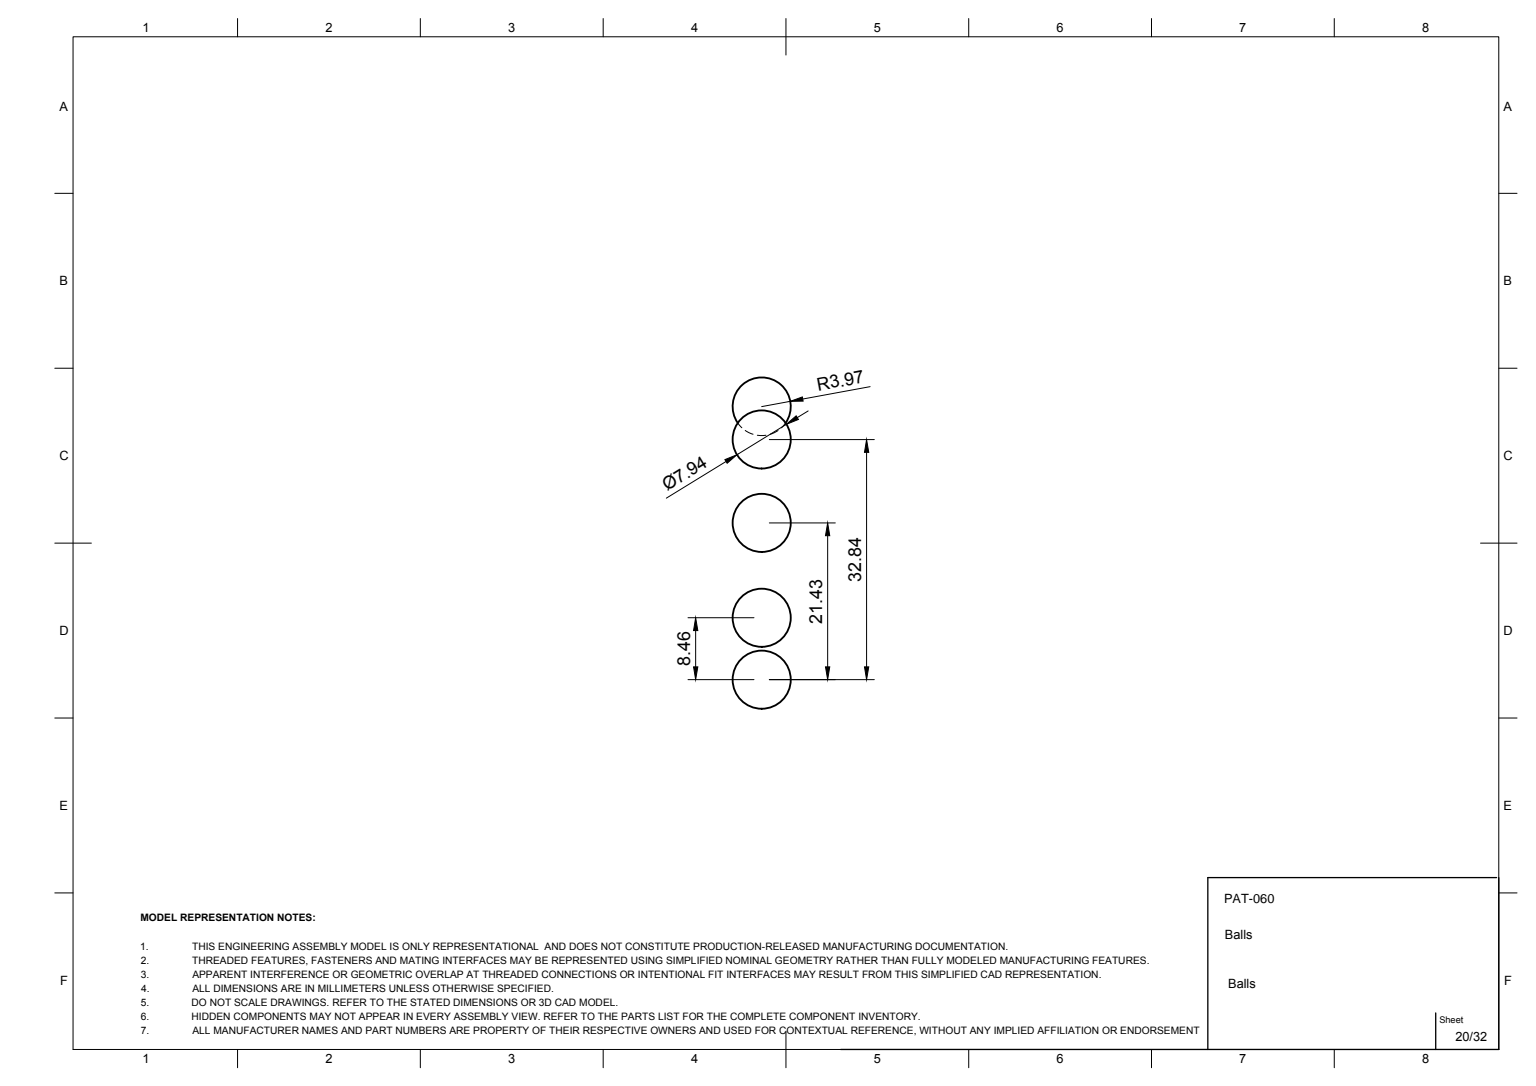
ISO-10303-21;
HEADER;
/* Generated by software containing ST-Developer
 * from STEP Tools, Inc. (www.steptools.com) 
 */

FILE_DESCRIPTION(
/* description */ ('Indexing fixture plate with plunger'),
/* implementation_level */ '2;1');

FILE_NAME(
/* name */ 'Balls.step',
/* time_stamp */ '2026-10-28T03:23:41-07:00',
/* author */ (''),
/* organization */ (''),
/* preprocessor_version */ 'ST-DEVELOPER v20.2',
/* originating_system */ 'Autodesk Translation Framework v15.17.0.0',
/* authorisation */ '');

FILE_SCHEMA (('AUTOMOTIVE_DESIGN { 1 0 10303 214 3 1 1 }'));
ENDSEC;

DATA;
#10=MECHANICAL_DESIGN_GEOMETRIC_PRESENTATION_REPRESENTATION('',(#332,#333,#334,#335,#336,#337,#338,#339,#340),#10020);
#195=SPHERICAL_SURFACE('',#5126,0.3969);
#196=SPHERICAL_SURFACE('',#5128,0.3969);
#197=SPHERICAL_SURFACE('',#5130,0.3969);
#198=SPHERICAL_SURFACE('',#5132,0.3969);
#199=SPHERICAL_SURFACE('',#5134,0.3969);
#200=SPHERICAL_SURFACE('',#5136,0.3969);
#201=SPHERICAL_SURFACE('',#5138,0.3969);
#202=SPHERICAL_SURFACE('',#5140,0.3969);
#203=SPHERICAL_SURFACE('',#5142,0.3969);
#278=SHAPE_REPRESENTATION_RELATIONSHIP('SRR','None',#10153,#305);
#305=ADVANCED_BREP_SHAPE_REPRESENTATION('',(#367,#368,#369,#370,#371,#372,
#373,#374,#375),#10006);
#332=STYLED_ITEM('',(#10368),#367);
#333=STYLED_ITEM('',(#10368),#368);
#334=STYLED_ITEM('',(#10368),#369);
#335=STYLED_ITEM('',(#10368),#370);
#336=STYLED_ITEM('',(#10368),#371);
#337=STYLED_ITEM('',(#10368),#372);
#338=STYLED_ITEM('',(#10368),#373);
#339=STYLED_ITEM('',(#10368),#374);
#340=STYLED_ITEM('',(#10368),#375);
#367=MANIFOLD_SOLID_BREP('Body1',#4587);
#368=MANIFOLD_SOLID_BREP('Body2',#4588);
#369=MANIFOLD_SOLID_BREP('Body3',#4589);
#370=MANIFOLD_SOLID_BREP('Body4',#4590);
#371=MANIFOLD_SOLID_BREP('Body5',#4591);
#372=MANIFOLD_SOLID_BREP('Body6',#4592);
#373=MANIFOLD_SOLID_BREP('Body7',#4593);
#374=MANIFOLD_SOLID_BREP('Body8',#4594);
#375=MANIFOLD_SOLID_BREP('Body9',#4595);
#772=FACE_OUTER_BOUND('',#1106,.T.);
#773=FACE_OUTER_BOUND('',#1107,.T.);
#774=FACE_OUTER_BOUND('',#1108,.T.);
#775=FACE_OUTER_BOUND('',#1109,.T.);
#776=FACE_OUTER_BOUND('',#1110,.T.);
#777=FACE_OUTER_BOUND('',#1111,.T.);
#778=FACE_OUTER_BOUND('',#1112,.T.);
#779=FACE_OUTER_BOUND('',#1113,.T.);
#780=FACE_OUTER_BOUND('',#1114,.T.);
#1106=EDGE_LOOP('',(#3435,#3436));
#1107=EDGE_LOOP('',(#3437,#3438));
#1108=EDGE_LOOP('',(#3439,#3440));
#1109=EDGE_LOOP('',(#3441,#3442));
#1110=EDGE_LOOP('',(#3443,#3444));
#1111=EDGE_LOOP('',(#3445,#3446));
#1112=EDGE_LOOP('',(#3447,#3448));
#1113=EDGE_LOOP('',(#3449,#3450));
#1114=EDGE_LOOP('',(#3451,#3452));
#1931=CIRCLE('',#5127,0.3969);
#1932=CIRCLE('',#5129,0.3969);
#1933=CIRCLE('',#5131,0.3969);
#1934=CIRCLE('',#5133,0.3969);
#1935=CIRCLE('',#5135,0.3969);
#1936=CIRCLE('',#5137,0.3969);
#1937=CIRCLE('',#5139,0.3969);
#1938=CIRCLE('',#5141,0.3969);
#1939=CIRCLE('',#5143,0.3969);
#2257=VERTEX_POINT('',#8670);
#2258=VERTEX_POINT('',#8671);
#2259=VERTEX_POINT('',#8674);
#2260=VERTEX_POINT('',#8675);
#2261=VERTEX_POINT('',#8678);
#2262=VERTEX_POINT('',#8679);
#2263=VERTEX_POINT('',#8682);
#2264=VERTEX_POINT('',#8683);
#2265=VERTEX_POINT('',#8686);
#2266=VERTEX_POINT('',#8687);
#2267=VERTEX_POINT('',#8690);
#2268=VERTEX_POINT('',#8691);
#2269=VERTEX_POINT('',#8694);
#2270=VERTEX_POINT('',#8695);
#2271=VERTEX_POINT('',#8698);
#2272=VERTEX_POINT('',#8699);
#2273=VERTEX_POINT('',#8702);
#2274=VERTEX_POINT('',#8703);
#2697=EDGE_CURVE('',#2257,#2258,#1931,.T.);
#2698=EDGE_CURVE('',#2259,#2260,#1932,.T.);
#2699=EDGE_CURVE('',#2261,#2262,#1933,.T.);
#2700=EDGE_CURVE('',#2263,#2264,#1934,.T.);
#2701=EDGE_CURVE('',#2265,#2266,#1935,.T.);
#2702=EDGE_CURVE('',#2267,#2268,#1936,.T.);
#2703=EDGE_CURVE('',#2269,#2270,#1937,.T.);
#2704=EDGE_CURVE('',#2271,#2272,#1938,.T.);
#2705=EDGE_CURVE('',#2273,#2274,#1939,.T.);
#3435=ORIENTED_EDGE('',*,*,#2697,.T.);
#3436=ORIENTED_EDGE('',*,*,#2697,.F.);
#3437=ORIENTED_EDGE('',*,*,#2698,.T.);
#3438=ORIENTED_EDGE('',*,*,#2698,.F.);
#3439=ORIENTED_EDGE('',*,*,#2699,.T.);
#3440=ORIENTED_EDGE('',*,*,#2699,.F.);
#3441=ORIENTED_EDGE('',*,*,#2700,.T.);
#3442=ORIENTED_EDGE('',*,*,#2700,.F.);
#3443=ORIENTED_EDGE('',*,*,#2701,.T.);
#3444=ORIENTED_EDGE('',*,*,#2701,.F.);
#3445=ORIENTED_EDGE('',*,*,#2702,.T.);
#3446=ORIENTED_EDGE('',*,*,#2702,.F.);
#3447=ORIENTED_EDGE('',*,*,#2703,.T.);
#3448=ORIENTED_EDGE('',*,*,#2703,.F.);
#3449=ORIENTED_EDGE('',*,*,#2704,.T.);
#3450=ORIENTED_EDGE('',*,*,#2704,.F.);
#3451=ORIENTED_EDGE('',*,*,#2705,.T.);
#3452=ORIENTED_EDGE('',*,*,#2705,.F.);
#4387=ADVANCED_FACE('',(#772),#195,.T.);
#4388=ADVANCED_FACE('',(#773),#196,.T.);
#4389=ADVANCED_FACE('',(#774),#197,.T.);
#4390=ADVANCED_FACE('',(#775),#198,.T.);
#4391=ADVANCED_FACE('',(#776),#199,.T.);
#4392=ADVANCED_FACE('',(#777),#200,.T.);
#4393=ADVANCED_FACE('',(#778),#201,.T.);
#4394=ADVANCED_FACE('',(#779),#202,.T.);
#4395=ADVANCED_FACE('',(#780),#203,.T.);
#4587=CLOSED_SHELL('',(#4387));
#4588=CLOSED_SHELL('',(#4388));
#4589=CLOSED_SHELL('',(#4389));
#4590=CLOSED_SHELL('',(#4390));
#4591=CLOSED_SHELL('',(#4391));
#4592=CLOSED_SHELL('',(#4392));
#4593=CLOSED_SHELL('',(#4393));
#4594=CLOSED_SHELL('',(#4394));
#4595=CLOSED_SHELL('',(#4395));
#5125=AXIS2_PLACEMENT_3D('',#8668,#6090,#6091);
#5126=AXIS2_PLACEMENT_3D('',#8669,#6092,#6093);
#5127=AXIS2_PLACEMENT_3D('',#8672,#6094,#6095);
#5128=AXIS2_PLACEMENT_3D('',#8673,#6096,#6097);
#5129=AXIS2_PLACEMENT_3D('',#8676,#6098,#6099);
#5130=AXIS2_PLACEMENT_3D('',#8677,#6100,#6101);
#5131=AXIS2_PLACEMENT_3D('',#8680,#6102,#6103);
#5132=AXIS2_PLACEMENT_3D('',#8681,#6104,#6105);
#5133=AXIS2_PLACEMENT_3D('',#8684,#6106,#6107);
#5134=AXIS2_PLACEMENT_3D('',#8685,#6108,#6109);
#5135=AXIS2_PLACEMENT_3D('',#8688,#6110,#6111);
#5136=AXIS2_PLACEMENT_3D('',#8689,#6112,#6113);
#5137=AXIS2_PLACEMENT_3D('',#8692,#6114,#6115);
#5138=AXIS2_PLACEMENT_3D('',#8693,#6116,#6117);
#5139=AXIS2_PLACEMENT_3D('',#8696,#6118,#6119);
#5140=AXIS2_PLACEMENT_3D('',#8697,#6120,#6121);
#5141=AXIS2_PLACEMENT_3D('',#8700,#6122,#6123);
#5142=AXIS2_PLACEMENT_3D('',#8701,#6124,#6125);
#5143=AXIS2_PLACEMENT_3D('',#8704,#6126,#6127);
#6090=DIRECTION('axis',(0.,0.,1.));
#6091=DIRECTION('refdir',(1.,0.,0.));
#6092=DIRECTION('center_axis',(0.,0.,1.));
#6093=DIRECTION('ref_axis',(1.,0.,0.));
#6094=DIRECTION('center_axis',(1.22464679914735E-16,-1.,0.));
#6095=DIRECTION('ref_axis',(-1.,-1.22464679914735E-16,0.));
#6096=DIRECTION('center_axis',(0.642787609686539,0.,0.766044443118978));
#6097=DIRECTION('ref_axis',(0.766044443118978,0.,-0.642787609686539));
#6098=DIRECTION('center_axis',(9.38133875270273E-17,-1.,-7.87187788734199E-17));
#6099=DIRECTION('ref_axis',(-0.766044443118978,-1.22464679914735E-16,0.642787609686539));
#6100=DIRECTION('center_axis',(0.984807753012208,0.,0.173648177666931));
#6101=DIRECTION('ref_axis',(0.17364817766693,0.,-0.984807753012208));
#6102=DIRECTION('center_axis',(2.12657684957577E-17,-1.,-1.2060416625019E-16));
#6103=DIRECTION('ref_axis',(-0.17364817766693,-1.22464679914735E-16,0.984807753012208));
#6104=DIRECTION('center_axis',(0.866025403784439,0.,-0.5));
#6105=DIRECTION('ref_axis',(-0.5,0.,-0.866025403784439));
#6106=DIRECTION('center_axis',(-6.12323399573676E-17,-1.,-1.06057523872491E-16));
#6107=DIRECTION('ref_axis',(0.5,-1.22464679914735E-16,0.866025403784439));
#6108=DIRECTION('center_axis',(0.342020143325669,0.,-0.939692620785908));
#6109=DIRECTION('ref_axis',(-0.939692620785908,0.,-0.342020143325669));
#6110=DIRECTION('center_axis',(-1.15079156022785E-16,-1.,-4.18853873767699E-17));
#6111=DIRECTION('ref_axis',(0.939692620785908,-1.22464679914735E-16,0.342020143325669));
#6112=DIRECTION('center_axis',(-0.342020143325669,0.,-0.939692620785908));
#6113=DIRECTION('ref_axis',(-0.939692620785909,0.,0.342020143325669));
#6114=DIRECTION('center_axis',(-1.15079156022785E-16,-1.,4.18853873767699E-17));
#6115=DIRECTION('ref_axis',(0.939692620785908,-1.22464679914735E-16,-0.342020143325669));
#6116=DIRECTION('center_axis',(-0.866025403784438,0.,-0.5));
#6117=DIRECTION('ref_axis',(-0.5,0.,0.866025403784438));
#6118=DIRECTION('center_axis',(-6.12323399573677E-17,-1.,1.06057523872491E-16));
#6119=DIRECTION('ref_axis',(0.5,-1.22464679914735E-16,-0.866025403784438));
#6120=DIRECTION('center_axis',(-0.984807753012208,0.,0.17364817766693));
#6121=DIRECTION('ref_axis',(0.17364817766693,0.,0.984807753012208));
#6122=DIRECTION('center_axis',(2.12657684957577E-17,-1.,1.2060416625019E-16));
#6123=DIRECTION('ref_axis',(-0.17364817766693,-1.22464679914735E-16,-0.984807753012208));
#6124=DIRECTION('center_axis',(-0.64278760968654,0.,0.766044443118978));
#6125=DIRECTION('ref_axis',(0.766044443118978,0.,0.64278760968654));
#6126=DIRECTION('center_axis',(9.38133875270273E-17,-1.,7.87187788734199E-17));
#6127=DIRECTION('ref_axis',(-0.766044443118978,-1.22464679914735E-16,-0.64278760968654));
#8668=CARTESIAN_POINT('',(0.,0.,0.));
#8669=CARTESIAN_POINT('Origin',(1.925,0.,0.));
#8670=CARTESIAN_POINT('',(1.925,-2.97627328869245E-33,0.3969));
#8671=CARTESIAN_POINT('',(1.925,-2.97627328869245E-33,-0.3969));
#8672=CARTESIAN_POINT('Origin',(1.925,0.,0.));
#8673=CARTESIAN_POINT('Origin',(1.47463555300403,0.,-1.23736614864659));
#8674=CARTESIAN_POINT('',(1.72975795528862,-2.97627328869245E-33,-0.933323109172666));
#8675=CARTESIAN_POINT('',(1.21951315071945,-2.97627328869245E-33,-1.54140918812051));
#8676=CARTESIAN_POINT('Origin',(1.47463555300403,0.,-1.23736614864659));
#8677=CARTESIAN_POINT('Origin',(0.334272742008841,0.,-1.8957549245485));
#8678=CARTESIAN_POINT('',(0.725142939179386,1.05214622327121E-34,-1.8268339628325));
#8679=CARTESIAN_POINT('',(-0.0565974551617042,-6.05776119971203E-33,-1.96467588626451));
#8680=CARTESIAN_POINT('Origin',(0.334272742008841,0.,-1.8957549245485));
#8681=CARTESIAN_POINT('Origin',(-0.9625,0.,-1.66709890228504));
#8682=CARTESIAN_POINT('',(-0.618774517237956,-2.97627328869245E-33,-1.86554890228504));
#8683=CARTESIAN_POINT('',(-1.30622548276204,-2.97627328869245E-33,-1.46864890228504));
#8684=CARTESIAN_POINT('Origin',(-0.9625,0.,-1.66709890228504));
#8685=CARTESIAN_POINT('Origin',(-1.80890829501287,0.,-0.658388775901913));
#8686=CARTESIAN_POINT('',(-1.67316050012692,1.05214622327121E-34,-1.03135277709184));
#8687=CARTESIAN_POINT('',(-1.94465608989883,-6.05776119971203E-33,-0.285424774711986));
#8688=CARTESIAN_POINT('Origin',(-1.80890829501287,0.,-0.658388775901913));
#8689=CARTESIAN_POINT('Origin',(-1.80890829501287,0.,0.658388775901912));
#8690=CARTESIAN_POINT('',(-1.94465608989883,-9.13924911073161E-33,0.285424774711985));
#8691=CARTESIAN_POINT('',(-1.67316050012692,3.1867025333467E-33,1.03135277709184));
#8692=CARTESIAN_POINT('Origin',(-1.80890829501287,0.,0.658388775901912));
#8693=CARTESIAN_POINT('Origin',(-0.962500000000001,0.,1.66709890228504));
#8694=CARTESIAN_POINT('',(-1.30622548276204,-2.97627328869245E-33,1.46864890228504));
#8695=CARTESIAN_POINT('',(-0.618774517237957,-2.97627328869245E-33,1.86554890228504));
#8696=CARTESIAN_POINT('Origin',(-0.962500000000001,0.,1.66709890228504));
#8697=CARTESIAN_POINT('Origin',(0.33427274200884,0.,1.8957549245485));
#8698=CARTESIAN_POINT('',(-0.0565974551617051,-2.97627328869245E-33,1.96467588626451));
#8699=CARTESIAN_POINT('',(0.725142939179386,-2.97627328869245E-33,1.8268339628325));
#8700=CARTESIAN_POINT('Origin',(0.33427274200884,0.,1.8957549245485));
#8701=CARTESIAN_POINT('Origin',(1.47463555300403,0.,1.23736614864659));
#8702=CARTESIAN_POINT('',(1.21951315071944,-6.05776119971203E-33,1.54140918812051));
#8703=CARTESIAN_POINT('',(1.72975795528862,1.05214622327122E-34,0.933323109172667));
#8704=CARTESIAN_POINT('Origin',(1.47463555300403,0.,1.23736614864659));
#9973=UNCERTAINTY_MEASURE_WITH_UNIT(LENGTH_MEASURE(0.001),#10021,
'DISTANCE_ACCURACY_VALUE',
'Maximum model space distance between geometric entities at asserted c
onnectivities');
#9987=UNCERTAINTY_MEASURE_WITH_UNIT(LENGTH_MEASURE(0.001),#10021,
'DISTANCE_ACCURACY_VALUE',
'Maximum model space distance between geometric entities at asserted c
onnectivities');
#10006=(
GEOMETRIC_REPRESENTATION_CONTEXT(3)
GLOBAL_UNCERTAINTY_ASSIGNED_CONTEXT((#9973))
GLOBAL_UNIT_ASSIGNED_CONTEXT((#10021,#10023,#10024))
REPRESENTATION_CONTEXT('','3D')
);
#10020=(
GEOMETRIC_REPRESENTATION_CONTEXT(3)
GLOBAL_UNCERTAINTY_ASSIGNED_CONTEXT((#9987))
GLOBAL_UNIT_ASSIGNED_CONTEXT((#10021,#10023,#10024))
REPRESENTATION_CONTEXT('','3D')
);
#10021=(
LENGTH_UNIT()
NAMED_UNIT(*)
SI_UNIT(.CENTI.,.METRE.)
);
#10023=(
NAMED_UNIT(*)
PLANE_ANGLE_UNIT()
SI_UNIT($,.RADIAN.)
);
#10024=(
NAMED_UNIT(*)
SI_UNIT($,.STERADIAN.)
SOLID_ANGLE_UNIT()
);
#10043=SHAPE_DEFINITION_REPRESENTATION(#10075,#10153);
#10075=PRODUCT_DEFINITION_SHAPE('',$,#10186);
#10153=SHAPE_REPRESENTATION('',(#5125),#10006);
#10167=PRODUCT_DEFINITION_CONTEXT('part definition',#10265,'design');
#10186=PRODUCT_DEFINITION('Balls','Balls',#10218,#10167);
#10218=PRODUCT_DEFINITION_FORMATION('',$,#10285);
#10265=APPLICATION_CONTEXT(
'Core Data for Automotive Mechanical Design Process');
#10266=PRODUCT_CONTEXT('part definition',#10265,'mechanical');
#10285=PRODUCT('Balls','Balls','Balls',(#10266));
#10362=COLOUR_RGB('Grey',0.48,0.52,0.57);
#10363=FILL_AREA_STYLE_COLOUR('',#10362);
#10364=FILL_AREA_STYLE('',(#10363));
#10365=SURFACE_STYLE_FILL_AREA(#10364);
#10366=SURFACE_SIDE_STYLE('',(#10365));
#10367=SURFACE_STYLE_USAGE(.BOTH.,#10366);
#10368=PRESENTATION_STYLE_ASSIGNMENT((#10367));
ENDSEC;
END-ISO-10303-21;
